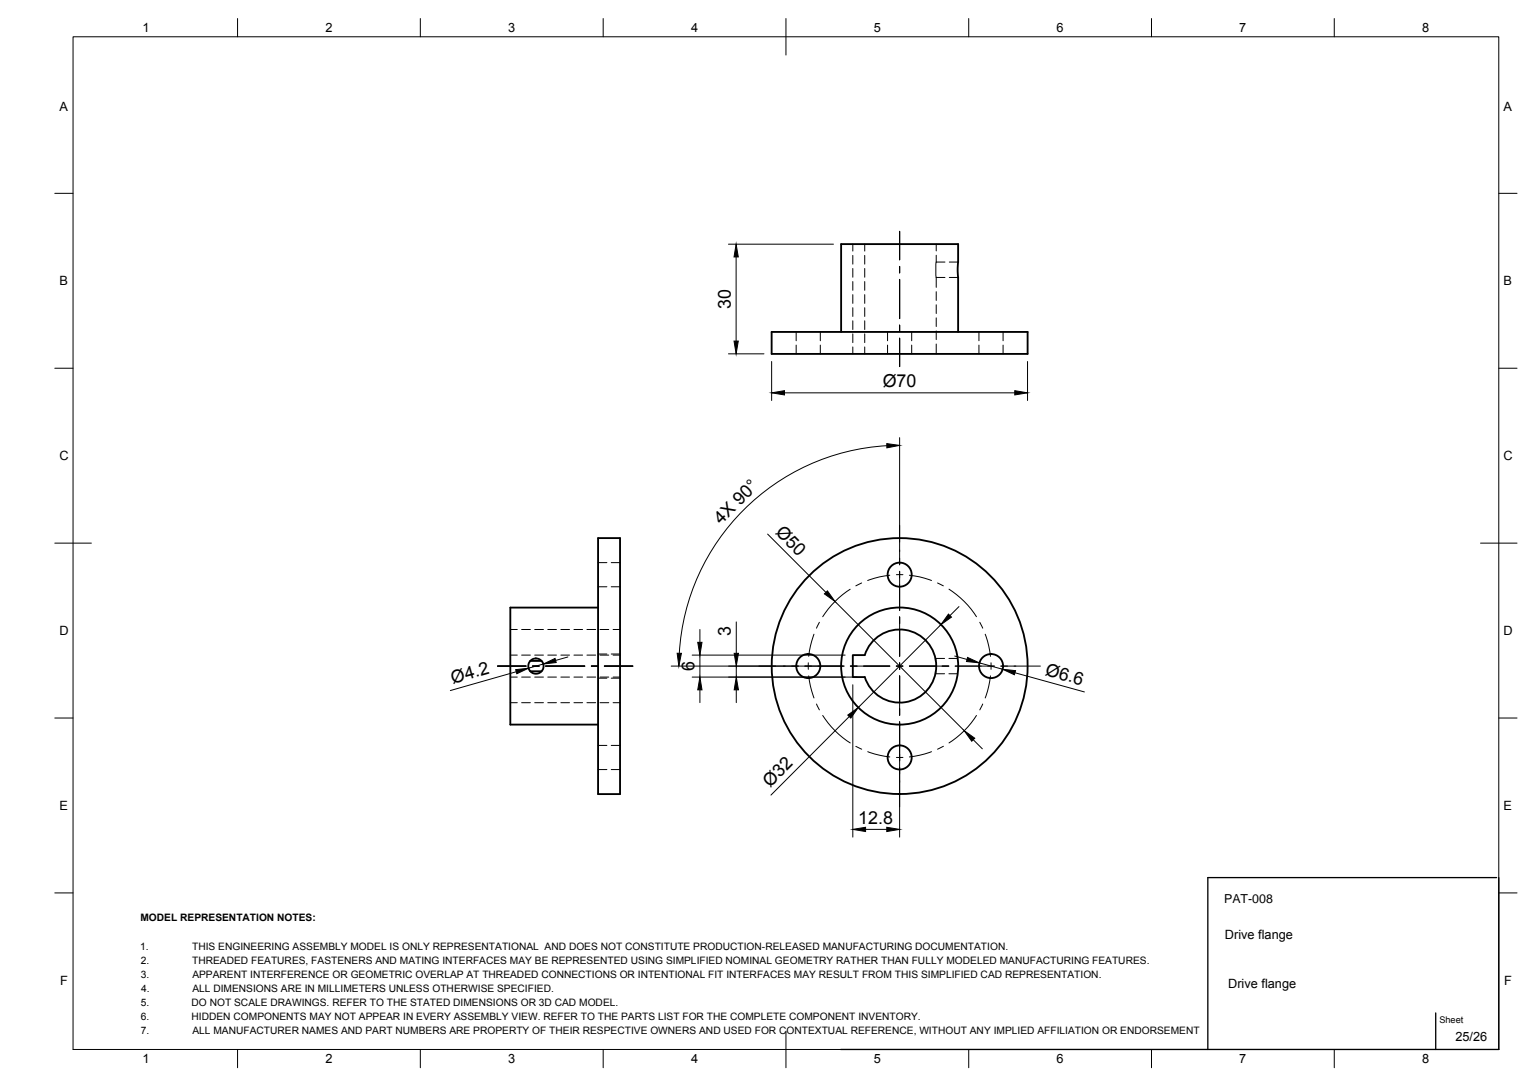
ISO-10303-21;
HEADER;
/* Generated by software containing ST-Developer
 * from STEP Tools, Inc. (www.steptools.com) 
 */

FILE_DESCRIPTION(
/* description */ ('Bearing housing with oil seal and end cap'),
/* implementation_level */ '2;1');

FILE_NAME(
/* name */ 'Drive flange.step',
/* time_stamp */ '2026-10-28T03:23:10-07:00',
/* author */ (''),
/* organization */ (''),
/* preprocessor_version */ 'ST-DEVELOPER v20.2',
/* originating_system */ 'Autodesk Translation Framework v15.17.0.0',
/* authorisation */ '');

FILE_SCHEMA (('AUTOMOTIVE_DESIGN { 1 0 10303 214 3 1 1 }'));
ENDSEC;

DATA;
#10=MECHANICAL_DESIGN_GEOMETRIC_PRESENTATION_REPRESENTATION('',(#285),#7871);
#181=B_SPLINE_CURVE_WITH_KNOTS('',3,(#7578,#7579,#7580,#7581,#7582,#7583,
#7584,#7585,#7586,#7587),.UNSPECIFIED.,.F.,.F.,(4,2,2,2,4),(0.803821788694075,
0.872950991853619,0.952307212900969,1.03166343394832,1.10079263710786),
 .UNSPECIFIED.);
#182=B_SPLINE_CURVE_WITH_KNOTS('',3,(#7593,#7594,#7595,#7596,#7597,#7598,
#7599,#7600,#7601,#7602,#7603,#7604,#7605,#7606,#7607,#7608,#7609,#7610),
 .UNSPECIFIED.,.F.,.F.,(4,2,2,2,2,2,2,2,4),(0.,0.0792028026112439,0.158405605222488,
0.237607602356377,0.316809599490266,0.396011596624156,0.475213593758045,
0.554416396369289,0.633619198980533),.UNSPECIFIED.);
#183=B_SPLINE_CURVE_WITH_KNOTS('',3,(#7611,#7612,#7613,#7614,#7615,#7616,
#7617,#7618,#7619,#7620,#7621,#7622,#7623,#7624,#7625,#7626,#7627,#7628),
 .UNSPECIFIED.,.F.,.F.,(4,2,2,2,2,2,2,2,4),(0.633619198980533,0.712822001591777,
0.792024804203021,0.87122680133691,0.9504287984708,1.02963079560469,1.10883279273858,
1.18803559534982,1.26723839796107),.UNSPECIFIED.);
#184=B_SPLINE_CURVE_WITH_KNOTS('',3,(#7631,#7632,#7633,#7634,#7635,#7636,
#7637,#7638,#7639,#7640),.UNSPECIFIED.,.F.,.F.,(4,2,2,2,4),(0.168950313426762,
0.238079516586307,0.317435737633656,0.396791958681006,0.465921161840551),
 .UNSPECIFIED.);
#235=SHAPE_REPRESENTATION_RELATIONSHIP('SRR','None',#7984,#256);
#256=ADVANCED_BREP_SHAPE_REPRESENTATION('',(#312),#7868);
#285=STYLED_ITEM('',(#8146),#312);
#312=MANIFOLD_SOLID_BREP('Body1',#4113);
#394=FACE_BOUND('',#1102,.T.);
#395=FACE_BOUND('',#1104,.T.);
#396=FACE_BOUND('',#1110,.T.);
#397=FACE_BOUND('',#1111,.T.);
#398=FACE_BOUND('',#1112,.T.);
#399=FACE_BOUND('',#1113,.T.);
#400=FACE_BOUND('',#1114,.T.);
#401=FACE_BOUND('',#1117,.T.);
#402=FACE_BOUND('',#1119,.T.);
#403=FACE_BOUND('',#1120,.T.);
#404=FACE_BOUND('',#1121,.T.);
#405=FACE_BOUND('',#1122,.T.);
#406=FACE_BOUND('',#1123,.T.);
#525=PLANE('',#4810);
#526=PLANE('',#4815);
#527=PLANE('',#4816);
#528=PLANE('',#4817);
#529=PLANE('',#4818);
#530=PLANE('',#4819);
#531=PLANE('',#4836);
#532=PLANE('',#4842);
#765=FACE_OUTER_BOUND('',#1095,.T.);
#766=FACE_OUTER_BOUND('',#1096,.T.);
#767=FACE_OUTER_BOUND('',#1097,.T.);
#768=FACE_OUTER_BOUND('',#1098,.T.);
#769=FACE_OUTER_BOUND('',#1099,.T.);
#770=FACE_OUTER_BOUND('',#1100,.T.);
#771=FACE_OUTER_BOUND('',#1101,.T.);
#772=FACE_OUTER_BOUND('',#1103,.T.);
#773=FACE_OUTER_BOUND('',#1105,.T.);
#774=FACE_OUTER_BOUND('',#1106,.T.);
#775=FACE_OUTER_BOUND('',#1107,.T.);
#776=FACE_OUTER_BOUND('',#1108,.T.);
#777=FACE_OUTER_BOUND('',#1109,.T.);
#778=FACE_OUTER_BOUND('',#1115,.T.);
#779=FACE_OUTER_BOUND('',#1116,.T.);
#780=FACE_OUTER_BOUND('',#1118,.T.);
#1095=EDGE_LOOP('',(#3581,#3582));
#1096=EDGE_LOOP('',(#3583,#3584,#3585,#3586,#3587,#3588,#3589,#3590,#3591));
#1097=EDGE_LOOP('',(#3592,#3593,#3594));
#1098=EDGE_LOOP('',(#3595,#3596,#3597,#3598));
#1099=EDGE_LOOP('',(#3599,#3600,#3601,#3602));
#1100=EDGE_LOOP('',(#3603,#3604,#3605,#3606));
#1101=EDGE_LOOP('',(#3607));
#1102=EDGE_LOOP('',(#3608,#3609,#3610,#3611));
#1103=EDGE_LOOP('',(#3612,#3613,#3614,#3615));
#1104=EDGE_LOOP('',(#3616,#3617,#3618,#3619));
#1105=EDGE_LOOP('',(#3620,#3621,#3622,#3623));
#1106=EDGE_LOOP('',(#3624,#3625,#3626,#3627));
#1107=EDGE_LOOP('',(#3628,#3629,#3630,#3631));
#1108=EDGE_LOOP('',(#3632,#3633,#3634,#3635));
#1109=EDGE_LOOP('',(#3636));
#1110=EDGE_LOOP('',(#3637));
#1111=EDGE_LOOP('',(#3638));
#1112=EDGE_LOOP('',(#3639));
#1113=EDGE_LOOP('',(#3640));
#1114=EDGE_LOOP('',(#3641));
#1115=EDGE_LOOP('',(#3642,#3643,#3644,#3645));
#1116=EDGE_LOOP('',(#3646,#3647,#3648,#3649));
#1117=EDGE_LOOP('',(#3650,#3651));
#1118=EDGE_LOOP('',(#3652));
#1119=EDGE_LOOP('',(#3653,#3654,#3655,#3656));
#1120=EDGE_LOOP('',(#3657));
#1121=EDGE_LOOP('',(#3658));
#1122=EDGE_LOOP('',(#3659));
#1123=EDGE_LOOP('',(#3660));
#1345=LINE('',#7574,#1607);
#1346=LINE('',#7591,#1608);
#1347=LINE('',#7642,#1609);
#1348=LINE('',#7646,#1610);
#1349=LINE('',#7648,#1611);
#1350=LINE('',#7650,#1612);
#1351=LINE('',#7651,#1613);
#1352=LINE('',#7654,#1614);
#1353=LINE('',#7656,#1615);
#1354=LINE('',#7657,#1616);
#1355=LINE('',#7660,#1617);
#1356=LINE('',#7662,#1618);
#1357=LINE('',#7663,#1619);
#1358=LINE('',#7674,#1620);
#1359=LINE('',#7680,#1621);
#1360=LINE('',#7686,#1622);
#1361=LINE('',#7692,#1623);
#1362=LINE('',#7701,#1624);
#1363=LINE('',#7704,#1625);
#1607=VECTOR('',#6004,1.);
#1608=VECTOR('',#6011,0.21);
#1609=VECTOR('',#6016,1.);
#1610=VECTOR('',#6019,1.);
#1611=VECTOR('',#6020,1.);
#1612=VECTOR('',#6021,1.);
#1613=VECTOR('',#6022,1.);
#1614=VECTOR('',#6025,1.);
#1615=VECTOR('',#6026,1.);
#1616=VECTOR('',#6027,1.);
#1617=VECTOR('',#6030,1.);
#1618=VECTOR('',#6031,1.);
#1619=VECTOR('',#6032,1.);
#1620=VECTOR('',#6047,0.33);
#1621=VECTOR('',#6054,0.33);
#1622=VECTOR('',#6061,0.33);
#1623=VECTOR('',#6068,0.33);
#1624=VECTOR('',#6079,3.5);
#1625=VECTOR('',#6084,1.6);
#1870=CIRCLE('',#4811,0.21);
#1871=CIRCLE('',#4813,0.21);
#1872=CIRCLE('',#4814,0.21);
#1873=CIRCLE('',#4820,1.6);
#1874=CIRCLE('',#4821,1.);
#1875=CIRCLE('',#4823,1.);
#1876=CIRCLE('',#4825,0.33);
#1877=CIRCLE('',#4826,0.33);
#1878=CIRCLE('',#4828,0.33);
#1879=CIRCLE('',#4829,0.33);
#1880=CIRCLE('',#4831,0.33);
#1881=CIRCLE('',#4832,0.33);
#1882=CIRCLE('',#4834,0.33);
#1883=CIRCLE('',#4835,0.33);
#1884=CIRCLE('',#4837,3.5);
#1885=CIRCLE('',#4838,1.6);
#1886=CIRCLE('',#4840,3.5);
#2176=VERTEX_POINT('',#7572);
#2177=VERTEX_POINT('',#7573);
#2178=VERTEX_POINT('',#7577);
#2179=VERTEX_POINT('',#7588);
#2180=VERTEX_POINT('',#7590);
#2181=VERTEX_POINT('',#7592);
#2182=VERTEX_POINT('',#7629);
#2183=VERTEX_POINT('',#7644);
#2184=VERTEX_POINT('',#7645);
#2185=VERTEX_POINT('',#7647);
#2186=VERTEX_POINT('',#7649);
#2187=VERTEX_POINT('',#7653);
#2188=VERTEX_POINT('',#7655);
#2189=VERTEX_POINT('',#7659);
#2190=VERTEX_POINT('',#7661);
#2191=VERTEX_POINT('',#7665);
#2192=VERTEX_POINT('',#7671);
#2193=VERTEX_POINT('',#7673);
#2194=VERTEX_POINT('',#7677);
#2195=VERTEX_POINT('',#7679);
#2196=VERTEX_POINT('',#7683);
#2197=VERTEX_POINT('',#7685);
#2198=VERTEX_POINT('',#7689);
#2199=VERTEX_POINT('',#7691);
#2200=VERTEX_POINT('',#7695);
#2201=VERTEX_POINT('',#7697);
#2202=VERTEX_POINT('',#7700);
#2654=EDGE_CURVE('',#2176,#2177,#1345,.T.);
#2655=EDGE_CURVE('',#2176,#2177,#1870,.T.);
#2656=EDGE_CURVE('',#2178,#2176,#181,.T.);
#2657=EDGE_CURVE('',#2179,#2178,#1871,.T.);
#2658=EDGE_CURVE('',#2179,#2180,#1346,.T.);
#2659=EDGE_CURVE('',#2181,#2180,#182,.T.);
#2660=EDGE_CURVE('',#2180,#2181,#183,.T.);
#2661=EDGE_CURVE('',#2182,#2179,#1872,.T.);
#2662=EDGE_CURVE('',#2177,#2182,#184,.T.);
#2663=EDGE_CURVE('',#2182,#2178,#1347,.T.);
#2664=EDGE_CURVE('',#2183,#2184,#1348,.T.);
#2665=EDGE_CURVE('',#2183,#2185,#1349,.T.);
#2666=EDGE_CURVE('',#2186,#2185,#1350,.T.);
#2667=EDGE_CURVE('',#2184,#2186,#1351,.T.);
#2668=EDGE_CURVE('',#2187,#2183,#1352,.T.);
#2669=EDGE_CURVE('',#2187,#2188,#1353,.T.);
#2670=EDGE_CURVE('',#2185,#2188,#1354,.T.);
#2671=EDGE_CURVE('',#2189,#2187,#1355,.T.);
#2672=EDGE_CURVE('',#2190,#2189,#1356,.T.);
#2673=EDGE_CURVE('',#2188,#2190,#1357,.T.);
#2674=EDGE_CURVE('',#2191,#2191,#1873,.T.);
#2675=EDGE_CURVE('',#2190,#2186,#1874,.T.);
#2676=EDGE_CURVE('',#2189,#2184,#1875,.T.);
#2677=EDGE_CURVE('',#2192,#2192,#1876,.T.);
#2678=EDGE_CURVE('',#2192,#2193,#1358,.T.);
#2679=EDGE_CURVE('',#2193,#2193,#1877,.T.);
#2680=EDGE_CURVE('',#2194,#2194,#1878,.T.);
#2681=EDGE_CURVE('',#2194,#2195,#1359,.T.);
#2682=EDGE_CURVE('',#2195,#2195,#1879,.T.);
#2683=EDGE_CURVE('',#2196,#2196,#1880,.T.);
#2684=EDGE_CURVE('',#2196,#2197,#1360,.T.);
#2685=EDGE_CURVE('',#2197,#2197,#1881,.T.);
#2686=EDGE_CURVE('',#2198,#2198,#1882,.T.);
#2687=EDGE_CURVE('',#2198,#2199,#1361,.T.);
#2688=EDGE_CURVE('',#2199,#2199,#1883,.T.);
#2689=EDGE_CURVE('',#2200,#2200,#1884,.T.);
#2690=EDGE_CURVE('',#2201,#2201,#1885,.T.);
#2691=EDGE_CURVE('',#2200,#2202,#1362,.T.);
#2692=EDGE_CURVE('',#2202,#2202,#1886,.T.);
#2693=EDGE_CURVE('',#2191,#2201,#1363,.T.);
#3581=ORIENTED_EDGE('',*,*,#2654,.F.);
#3582=ORIENTED_EDGE('',*,*,#2655,.T.);
#3583=ORIENTED_EDGE('',*,*,#2656,.F.);
#3584=ORIENTED_EDGE('',*,*,#2657,.F.);
#3585=ORIENTED_EDGE('',*,*,#2658,.T.);
#3586=ORIENTED_EDGE('',*,*,#2659,.F.);
#3587=ORIENTED_EDGE('',*,*,#2660,.F.);
#3588=ORIENTED_EDGE('',*,*,#2658,.F.);
#3589=ORIENTED_EDGE('',*,*,#2661,.F.);
#3590=ORIENTED_EDGE('',*,*,#2662,.F.);
#3591=ORIENTED_EDGE('',*,*,#2655,.F.);
#3592=ORIENTED_EDGE('',*,*,#2663,.F.);
#3593=ORIENTED_EDGE('',*,*,#2661,.T.);
#3594=ORIENTED_EDGE('',*,*,#2657,.T.);
#3595=ORIENTED_EDGE('',*,*,#2664,.F.);
#3596=ORIENTED_EDGE('',*,*,#2665,.T.);
#3597=ORIENTED_EDGE('',*,*,#2666,.F.);
#3598=ORIENTED_EDGE('',*,*,#2667,.F.);
#3599=ORIENTED_EDGE('',*,*,#2668,.F.);
#3600=ORIENTED_EDGE('',*,*,#2669,.T.);
#3601=ORIENTED_EDGE('',*,*,#2670,.F.);
#3602=ORIENTED_EDGE('',*,*,#2665,.F.);
#3603=ORIENTED_EDGE('',*,*,#2671,.F.);
#3604=ORIENTED_EDGE('',*,*,#2672,.F.);
#3605=ORIENTED_EDGE('',*,*,#2673,.F.);
#3606=ORIENTED_EDGE('',*,*,#2669,.F.);
#3607=ORIENTED_EDGE('',*,*,#2674,.T.);
#3608=ORIENTED_EDGE('',*,*,#2666,.T.);
#3609=ORIENTED_EDGE('',*,*,#2670,.T.);
#3610=ORIENTED_EDGE('',*,*,#2673,.T.);
#3611=ORIENTED_EDGE('',*,*,#2675,.T.);
#3612=ORIENTED_EDGE('',*,*,#2667,.T.);
#3613=ORIENTED_EDGE('',*,*,#2675,.F.);
#3614=ORIENTED_EDGE('',*,*,#2672,.T.);
#3615=ORIENTED_EDGE('',*,*,#2676,.T.);
#3616=ORIENTED_EDGE('',*,*,#2662,.T.);
#3617=ORIENTED_EDGE('',*,*,#2663,.T.);
#3618=ORIENTED_EDGE('',*,*,#2656,.T.);
#3619=ORIENTED_EDGE('',*,*,#2654,.T.);
#3620=ORIENTED_EDGE('',*,*,#2677,.F.);
#3621=ORIENTED_EDGE('',*,*,#2678,.T.);
#3622=ORIENTED_EDGE('',*,*,#2679,.F.);
#3623=ORIENTED_EDGE('',*,*,#2678,.F.);
#3624=ORIENTED_EDGE('',*,*,#2680,.F.);
#3625=ORIENTED_EDGE('',*,*,#2681,.T.);
#3626=ORIENTED_EDGE('',*,*,#2682,.F.);
#3627=ORIENTED_EDGE('',*,*,#2681,.F.);
#3628=ORIENTED_EDGE('',*,*,#2683,.F.);
#3629=ORIENTED_EDGE('',*,*,#2684,.T.);
#3630=ORIENTED_EDGE('',*,*,#2685,.F.);
#3631=ORIENTED_EDGE('',*,*,#2684,.F.);
#3632=ORIENTED_EDGE('',*,*,#2686,.F.);
#3633=ORIENTED_EDGE('',*,*,#2687,.T.);
#3634=ORIENTED_EDGE('',*,*,#2688,.F.);
#3635=ORIENTED_EDGE('',*,*,#2687,.F.);
#3636=ORIENTED_EDGE('',*,*,#2689,.T.);
#3637=ORIENTED_EDGE('',*,*,#2690,.F.);
#3638=ORIENTED_EDGE('',*,*,#2688,.T.);
#3639=ORIENTED_EDGE('',*,*,#2685,.T.);
#3640=ORIENTED_EDGE('',*,*,#2682,.T.);
#3641=ORIENTED_EDGE('',*,*,#2679,.T.);
#3642=ORIENTED_EDGE('',*,*,#2689,.F.);
#3643=ORIENTED_EDGE('',*,*,#2691,.T.);
#3644=ORIENTED_EDGE('',*,*,#2692,.T.);
#3645=ORIENTED_EDGE('',*,*,#2691,.F.);
#3646=ORIENTED_EDGE('',*,*,#2674,.F.);
#3647=ORIENTED_EDGE('',*,*,#2693,.T.);
#3648=ORIENTED_EDGE('',*,*,#2690,.T.);
#3649=ORIENTED_EDGE('',*,*,#2693,.F.);
#3650=ORIENTED_EDGE('',*,*,#2659,.T.);
#3651=ORIENTED_EDGE('',*,*,#2660,.T.);
#3652=ORIENTED_EDGE('',*,*,#2692,.F.);
#3653=ORIENTED_EDGE('',*,*,#2664,.T.);
#3654=ORIENTED_EDGE('',*,*,#2676,.F.);
#3655=ORIENTED_EDGE('',*,*,#2671,.T.);
#3656=ORIENTED_EDGE('',*,*,#2668,.T.);
#3657=ORIENTED_EDGE('',*,*,#2686,.T.);
#3658=ORIENTED_EDGE('',*,*,#2683,.T.);
#3659=ORIENTED_EDGE('',*,*,#2680,.T.);
#3660=ORIENTED_EDGE('',*,*,#2677,.T.);
#3825=CYLINDRICAL_SURFACE('',#4812,0.21);
#3826=CYLINDRICAL_SURFACE('',#4822,1.);
#3827=CYLINDRICAL_SURFACE('',#4824,0.33);
#3828=CYLINDRICAL_SURFACE('',#4827,0.33);
#3829=CYLINDRICAL_SURFACE('',#4830,0.33);
#3830=CYLINDRICAL_SURFACE('',#4833,0.33);
#3831=CYLINDRICAL_SURFACE('',#4839,3.5);
#3832=CYLINDRICAL_SURFACE('',#4841,1.6);
#4047=ADVANCED_FACE('',(#765),#525,.T.);
#4048=ADVANCED_FACE('',(#766),#3825,.F.);
#4049=ADVANCED_FACE('',(#767),#526,.T.);
#4050=ADVANCED_FACE('',(#768),#527,.F.);
#4051=ADVANCED_FACE('',(#769),#528,.F.);
#4052=ADVANCED_FACE('',(#770),#529,.F.);
#4053=ADVANCED_FACE('',(#771,#394),#530,.T.);
#4054=ADVANCED_FACE('',(#772,#395),#3826,.F.);
#4055=ADVANCED_FACE('',(#773),#3827,.F.);
#4056=ADVANCED_FACE('',(#774),#3828,.F.);
#4057=ADVANCED_FACE('',(#775),#3829,.F.);
#4058=ADVANCED_FACE('',(#776),#3830,.F.);
#4059=ADVANCED_FACE('',(#777,#396,#397,#398,#399,#400),#531,.T.);
#4060=ADVANCED_FACE('',(#778),#3831,.T.);
#4061=ADVANCED_FACE('',(#779,#401),#3832,.T.);
#4062=ADVANCED_FACE('',(#780,#402,#403,#404,#405,#406),#532,.F.);
#4113=CLOSED_SHELL('',(#4047,#4048,#4049,#4050,#4051,#4052,#4053,#4054,
#4055,#4056,#4057,#4058,#4059,#4060,#4061,#4062));
#4809=AXIS2_PLACEMENT_3D('',#7570,#6000,#6001);
#4810=AXIS2_PLACEMENT_3D('',#7571,#6002,#6003);
#4811=AXIS2_PLACEMENT_3D('',#7575,#6005,#6006);
#4812=AXIS2_PLACEMENT_3D('',#7576,#6007,#6008);
#4813=AXIS2_PLACEMENT_3D('',#7589,#6009,#6010);
#4814=AXIS2_PLACEMENT_3D('',#7630,#6012,#6013);
#4815=AXIS2_PLACEMENT_3D('',#7641,#6014,#6015);
#4816=AXIS2_PLACEMENT_3D('',#7643,#6017,#6018);
#4817=AXIS2_PLACEMENT_3D('',#7652,#6023,#6024);
#4818=AXIS2_PLACEMENT_3D('',#7658,#6028,#6029);
#4819=AXIS2_PLACEMENT_3D('',#7664,#6033,#6034);
#4820=AXIS2_PLACEMENT_3D('',#7666,#6035,#6036);
#4821=AXIS2_PLACEMENT_3D('',#7667,#6037,#6038);
#4822=AXIS2_PLACEMENT_3D('',#7668,#6039,#6040);
#4823=AXIS2_PLACEMENT_3D('',#7669,#6041,#6042);
#4824=AXIS2_PLACEMENT_3D('',#7670,#6043,#6044);
#4825=AXIS2_PLACEMENT_3D('',#7672,#6045,#6046);
#4826=AXIS2_PLACEMENT_3D('',#7675,#6048,#6049);
#4827=AXIS2_PLACEMENT_3D('',#7676,#6050,#6051);
#4828=AXIS2_PLACEMENT_3D('',#7678,#6052,#6053);
#4829=AXIS2_PLACEMENT_3D('',#7681,#6055,#6056);
#4830=AXIS2_PLACEMENT_3D('',#7682,#6057,#6058);
#4831=AXIS2_PLACEMENT_3D('',#7684,#6059,#6060);
#4832=AXIS2_PLACEMENT_3D('',#7687,#6062,#6063);
#4833=AXIS2_PLACEMENT_3D('',#7688,#6064,#6065);
#4834=AXIS2_PLACEMENT_3D('',#7690,#6066,#6067);
#4835=AXIS2_PLACEMENT_3D('',#7693,#6069,#6070);
#4836=AXIS2_PLACEMENT_3D('',#7694,#6071,#6072);
#4837=AXIS2_PLACEMENT_3D('',#7696,#6073,#6074);
#4838=AXIS2_PLACEMENT_3D('',#7698,#6075,#6076);
#4839=AXIS2_PLACEMENT_3D('',#7699,#6077,#6078);
#4840=AXIS2_PLACEMENT_3D('',#7702,#6080,#6081);
#4841=AXIS2_PLACEMENT_3D('',#7703,#6082,#6083);
#4842=AXIS2_PLACEMENT_3D('',#7705,#6085,#6086);
#6000=DIRECTION('axis',(0.,0.,1.));
#6001=DIRECTION('refdir',(1.,0.,0.));
#6002=DIRECTION('center_axis',(0.,0.,1.));
#6003=DIRECTION('ref_axis',(1.,0.,0.));
#6004=DIRECTION('',(0.,1.,0.));
#6005=DIRECTION('center_axis',(0.,0.,1.));
#6006=DIRECTION('ref_axis',(1.,0.,0.));
#6007=DIRECTION('center_axis',(0.,0.,1.));
#6008=DIRECTION('ref_axis',(1.,0.,0.));
#6009=DIRECTION('center_axis',(0.,0.,1.));
#6010=DIRECTION('ref_axis',(1.,0.,0.));
#6011=DIRECTION('',(0.,0.,1.));
#6012=DIRECTION('center_axis',(0.,0.,1.));
#6013=DIRECTION('ref_axis',(1.,0.,0.));
#6014=DIRECTION('center_axis',(0.,0.,1.));
#6015=DIRECTION('ref_axis',(1.,0.,0.));
#6016=DIRECTION('',(0.,-1.,0.));
#6017=DIRECTION('center_axis',(-1.,0.,0.));
#6018=DIRECTION('ref_axis',(0.,0.,1.));
#6019=DIRECTION('',(0.,0.,1.));
#6020=DIRECTION('',(0.,1.,0.));
#6021=DIRECTION('',(0.,0.,-1.));
#6022=DIRECTION('',(0.,1.,0.));
#6023=DIRECTION('center_axis',(0.,0.,-1.));
#6024=DIRECTION('ref_axis',(-1.,0.,0.));
#6025=DIRECTION('',(-1.,0.,0.));
#6026=DIRECTION('',(0.,1.,0.));
#6027=DIRECTION('',(1.,0.,0.));
#6028=DIRECTION('center_axis',(1.,0.,0.));
#6029=DIRECTION('ref_axis',(0.,0.,-1.));
#6030=DIRECTION('',(0.,0.,-1.));
#6031=DIRECTION('',(0.,-1.,0.));
#6032=DIRECTION('',(0.,0.,1.));
#6033=DIRECTION('center_axis',(0.,1.,0.));
#6034=DIRECTION('ref_axis',(1.,0.,0.));
#6035=DIRECTION('center_axis',(0.,1.,0.));
#6036=DIRECTION('ref_axis',(1.,0.,0.));
#6037=DIRECTION('center_axis',(0.,-1.,0.));
#6038=DIRECTION('ref_axis',(1.,0.,0.));
#6039=DIRECTION('center_axis',(0.,1.,0.));
#6040=DIRECTION('ref_axis',(-1.83697019872103E-16,0.,1.));
#6041=DIRECTION('center_axis',(0.,-1.,0.));
#6042=DIRECTION('ref_axis',(1.,0.,0.));
#6043=DIRECTION('center_axis',(0.,1.,0.));
#6044=DIRECTION('ref_axis',(1.,0.,0.));
#6045=DIRECTION('center_axis',(0.,1.,0.));
#6046=DIRECTION('ref_axis',(1.,0.,0.));
#6047=DIRECTION('',(0.,1.,0.));
#6048=DIRECTION('center_axis',(0.,-1.,0.));
#6049=DIRECTION('ref_axis',(1.,0.,0.));
#6050=DIRECTION('center_axis',(0.,1.,0.));
#6051=DIRECTION('ref_axis',(1.,0.,0.));
#6052=DIRECTION('center_axis',(0.,1.,0.));
#6053=DIRECTION('ref_axis',(1.,0.,0.));
#6054=DIRECTION('',(0.,1.,0.));
#6055=DIRECTION('center_axis',(0.,-1.,0.));
#6056=DIRECTION('ref_axis',(1.,0.,0.));
#6057=DIRECTION('center_axis',(0.,1.,0.));
#6058=DIRECTION('ref_axis',(1.,0.,0.));
#6059=DIRECTION('center_axis',(0.,1.,0.));
#6060=DIRECTION('ref_axis',(1.,0.,0.));
#6061=DIRECTION('',(0.,1.,0.));
#6062=DIRECTION('center_axis',(0.,-1.,0.));
#6063=DIRECTION('ref_axis',(1.,0.,0.));
#6064=DIRECTION('center_axis',(0.,1.,0.));
#6065=DIRECTION('ref_axis',(1.,0.,0.));
#6066=DIRECTION('center_axis',(0.,1.,0.));
#6067=DIRECTION('ref_axis',(1.,0.,0.));
#6068=DIRECTION('',(0.,1.,0.));
#6069=DIRECTION('center_axis',(0.,-1.,0.));
#6070=DIRECTION('ref_axis',(1.,0.,0.));
#6071=DIRECTION('center_axis',(0.,1.,0.));
#6072=DIRECTION('ref_axis',(1.,0.,0.));
#6073=DIRECTION('center_axis',(0.,1.,0.));
#6074=DIRECTION('ref_axis',(1.,0.,0.));
#6075=DIRECTION('center_axis',(0.,1.,0.));
#6076=DIRECTION('ref_axis',(1.,0.,0.));
#6077=DIRECTION('center_axis',(0.,1.,0.));
#6078=DIRECTION('ref_axis',(1.,0.,0.));
#6079=DIRECTION('',(0.,-1.,0.));
#6080=DIRECTION('center_axis',(0.,1.,0.));
#6081=DIRECTION('ref_axis',(1.,0.,0.));
#6082=DIRECTION('center_axis',(0.,1.,0.));
#6083=DIRECTION('ref_axis',(1.,0.,0.));
#6084=DIRECTION('',(0.,-1.,0.));
#6085=DIRECTION('center_axis',(0.,1.,0.));
#6086=DIRECTION('ref_axis',(1.,0.,0.));
#7570=CARTESIAN_POINT('',(0.,0.,0.));
#7571=CARTESIAN_POINT('Origin',(0.,-1.2,5.49));
#7572=CARTESIAN_POINT('',(0.141067359796657,-1.35556349186104,5.49));
#7573=CARTESIAN_POINT('',(0.141067359796657,-1.04443650813896,5.49));
#7574=CARTESIAN_POINT('',(0.141067359796657,-3.5,5.49));
#7575=CARTESIAN_POINT('Origin',(0.,-1.2,5.49));
#7576=CARTESIAN_POINT('Origin',(0.,-1.2,5.49));
#7577=CARTESIAN_POINT('',(-0.141067359796657,-1.35556349186104,5.49));
#7578=CARTESIAN_POINT('Ctrl Pts',(-0.141067359796657,-1.35556349186104,
5.49));
#7579=CARTESIAN_POINT('Ctrl Pts',(-0.123818356698224,-1.3712051523632,5.49245784982446));
#7580=CARTESIAN_POINT('Ctrl Pts',(-0.102998643109699,-1.38462404333102,
5.49493819304946));
#7581=CARTESIAN_POINT('Ctrl Pts',(-0.054614114398353,-1.40469746372443,
5.49884449237241));
#7582=CARTESIAN_POINT('Ctrl Pts',(-0.0264520736824499,-1.41,5.5));
#7583=CARTESIAN_POINT('Ctrl Pts',(0.0264520736824498,-1.41,5.5));
#7584=CARTESIAN_POINT('Ctrl Pts',(0.0546141143983528,-1.40469746372443,
5.49884449237241));
#7585=CARTESIAN_POINT('Ctrl Pts',(0.102998643109699,-1.38462404333102,5.49493819304946));
#7586=CARTESIAN_POINT('Ctrl Pts',(0.123818356698224,-1.3712051523632,5.49245784982446));
#7587=CARTESIAN_POINT('Ctrl Pts',(0.141067359796657,-1.35556349186104,5.49));
#7588=CARTESIAN_POINT('',(-0.21,-1.2,5.49));
#7589=CARTESIAN_POINT('Origin',(0.,-1.2,5.49));
#7590=CARTESIAN_POINT('',(-0.21,-1.2,6.08615888233178));
#7591=CARTESIAN_POINT('',(-0.21,-1.2,5.49));
#7592=CARTESIAN_POINT('',(0.21,-1.2,6.08615888233178));
#7593=CARTESIAN_POINT('Ctrl Pts',(0.21,-1.2,6.08615888233178));
#7594=CARTESIAN_POINT('Ctrl Pts',(0.21,-1.22640093420375,6.08615888233178));
#7595=CARTESIAN_POINT('Ctrl Pts',(0.20471752266132,-1.25454055536511,6.08688606295397));
#7596=CARTESIAN_POINT('Ctrl Pts',(0.183276841782292,-1.3062710523005,6.08950502964782));
#7597=CARTESIAN_POINT('Ctrl Pts',(0.167120287247804,-1.32986456085055,6.09135816887013));
#7598=CARTESIAN_POINT('Ctrl Pts',(0.129864750292352,-1.367120097806,6.09483075953278));
#7599=CARTESIAN_POINT('Ctrl Pts',(0.106271159541076,-1.38327680083123,6.09667690933009));
#7600=CARTESIAN_POINT('Ctrl Pts',(0.0545403836274685,-1.4047175903444,6.09927985626981));
#7601=CARTESIAN_POINT('Ctrl Pts',(0.0264006657112964,-1.41,6.1));
#7602=CARTESIAN_POINT('Ctrl Pts',(-0.0264006657112964,-1.41,6.1));
#7603=CARTESIAN_POINT('Ctrl Pts',(-0.0545403836274684,-1.4047175903444,
6.09927985626981));
#7604=CARTESIAN_POINT('Ctrl Pts',(-0.106271159541075,-1.38327680083123,
6.09667690933009));
#7605=CARTESIAN_POINT('Ctrl Pts',(-0.129864750292352,-1.367120097806,6.09483075953278));
#7606=CARTESIAN_POINT('Ctrl Pts',(-0.167120287247804,-1.32986456085055,
6.09135816887013));
#7607=CARTESIAN_POINT('Ctrl Pts',(-0.183276841782292,-1.3062710523005,6.08950502964782));
#7608=CARTESIAN_POINT('Ctrl Pts',(-0.20471752266132,-1.25454055536511,6.08688606295397));
#7609=CARTESIAN_POINT('Ctrl Pts',(-0.21,-1.22640093420375,6.08615888233178));
#7610=CARTESIAN_POINT('Ctrl Pts',(-0.21,-1.2,6.08615888233178));
#7611=CARTESIAN_POINT('Ctrl Pts',(-0.21,-1.2,6.08615888233178));
#7612=CARTESIAN_POINT('Ctrl Pts',(-0.21,-1.17359906579625,6.08615888233178));
#7613=CARTESIAN_POINT('Ctrl Pts',(-0.20471752266132,-1.14545944463489,6.08688606295397));
#7614=CARTESIAN_POINT('Ctrl Pts',(-0.183276841782292,-1.0937289476995,6.08950502964782));
#7615=CARTESIAN_POINT('Ctrl Pts',(-0.167120287247804,-1.07013543914945,
6.09135816887013));
#7616=CARTESIAN_POINT('Ctrl Pts',(-0.129864750292352,-1.032879902194,6.09483075953278));
#7617=CARTESIAN_POINT('Ctrl Pts',(-0.106271159541076,-1.01672319916877,
6.09667690933009));
#7618=CARTESIAN_POINT('Ctrl Pts',(-0.0545403836274687,-0.995282409655599,
6.09927985626981));
#7619=CARTESIAN_POINT('Ctrl Pts',(-0.0264006657112964,-0.99,6.1));
#7620=CARTESIAN_POINT('Ctrl Pts',(0.0264006657112964,-0.99,6.1));
#7621=CARTESIAN_POINT('Ctrl Pts',(0.0545403836274687,-0.995282409655599,
6.09927985626981));
#7622=CARTESIAN_POINT('Ctrl Pts',(0.106271159541076,-1.01672319916877,6.09667690933009));
#7623=CARTESIAN_POINT('Ctrl Pts',(0.129864750292352,-1.032879902194,6.09483075953278));
#7624=CARTESIAN_POINT('Ctrl Pts',(0.167120287247804,-1.07013543914945,6.09135816887013));
#7625=CARTESIAN_POINT('Ctrl Pts',(0.183276841782292,-1.0937289476995,6.08950502964782));
#7626=CARTESIAN_POINT('Ctrl Pts',(0.20471752266132,-1.14545944463489,6.08688606295397));
#7627=CARTESIAN_POINT('Ctrl Pts',(0.21,-1.17359906579625,6.08615888233178));
#7628=CARTESIAN_POINT('Ctrl Pts',(0.21,-1.2,6.08615888233178));
#7629=CARTESIAN_POINT('',(-0.141067359796657,-1.04443650813896,5.49));
#7630=CARTESIAN_POINT('Origin',(0.,-1.2,5.49));
#7631=CARTESIAN_POINT('Ctrl Pts',(0.141067359796657,-1.04443650813896,5.49));
#7632=CARTESIAN_POINT('Ctrl Pts',(0.123818356698224,-1.0287948476368,5.49245784982446));
#7633=CARTESIAN_POINT('Ctrl Pts',(0.102998643109699,-1.01537595666898,5.49493819304946));
#7634=CARTESIAN_POINT('Ctrl Pts',(0.0546141143983531,-0.995302536275572,
5.49884449237241));
#7635=CARTESIAN_POINT('Ctrl Pts',(0.0264520736824498,-0.99,5.5));
#7636=CARTESIAN_POINT('Ctrl Pts',(-0.0264520736824498,-0.99,5.5));
#7637=CARTESIAN_POINT('Ctrl Pts',(-0.054614114398353,-0.995302536275572,
5.49884449237241));
#7638=CARTESIAN_POINT('Ctrl Pts',(-0.102998643109699,-1.01537595666898,
5.49493819304946));
#7639=CARTESIAN_POINT('Ctrl Pts',(-0.123818356698224,-1.0287948476368,5.49245784982446));
#7640=CARTESIAN_POINT('Ctrl Pts',(-0.141067359796657,-1.04443650813896,
5.49));
#7641=CARTESIAN_POINT('Origin',(0.,-1.2,5.49));
#7642=CARTESIAN_POINT('',(-0.141067359796657,-3.5,5.49));
#7643=CARTESIAN_POINT('Origin',(-0.3,-3.6,3.22));
#7644=CARTESIAN_POINT('',(-0.3,-3.5,3.22));
#7645=CARTESIAN_POINT('',(-0.3,-3.5,3.54606079858305));
#7646=CARTESIAN_POINT('',(-0.3,-3.5,3.86));
#7647=CARTESIAN_POINT('',(-0.3,-0.5,3.22));
#7648=CARTESIAN_POINT('',(-0.3,-3.6,3.22));
#7649=CARTESIAN_POINT('',(-0.3,-0.5,3.54606079858305));
#7650=CARTESIAN_POINT('',(-0.3,-0.5,3.86));
#7651=CARTESIAN_POINT('',(-0.3,-3.5,3.54606079858305));
#7652=CARTESIAN_POINT('Origin',(0.3,-3.6,3.22));
#7653=CARTESIAN_POINT('',(0.3,-3.5,3.22));
#7654=CARTESIAN_POINT('',(0.15,-3.5,3.22));
#7655=CARTESIAN_POINT('',(0.3,-0.5,3.22));
#7656=CARTESIAN_POINT('',(0.3,-3.6,3.22));
#7657=CARTESIAN_POINT('',(0.15,-0.5,3.22));
#7658=CARTESIAN_POINT('Origin',(0.3,-3.6,4.5));
#7659=CARTESIAN_POINT('',(0.3,-3.5,3.54606079858305));
#7660=CARTESIAN_POINT('',(0.3,-3.5,4.5));
#7661=CARTESIAN_POINT('',(0.3,-0.5,3.54606079858305));
#7662=CARTESIAN_POINT('',(0.3,-3.5,3.54606079858305));
#7663=CARTESIAN_POINT('',(0.3,-0.5,4.5));
#7664=CARTESIAN_POINT('Origin',(0.,-0.5,4.5));
#7665=CARTESIAN_POINT('',(-1.6,-0.5,4.5));
#7666=CARTESIAN_POINT('Origin',(0.,-0.5,4.5));
#7667=CARTESIAN_POINT('Origin',(0.,-0.5,4.5));
#7668=CARTESIAN_POINT('Origin',(0.,-3.5,4.5));
#7669=CARTESIAN_POINT('Origin',(0.,-3.5,4.5));
#7670=CARTESIAN_POINT('Origin',(-2.5,-3.6,4.5));
#7671=CARTESIAN_POINT('',(-2.83,-3.5,4.5));
#7672=CARTESIAN_POINT('Origin',(-2.5,-3.5,4.5));
#7673=CARTESIAN_POINT('',(-2.83,-2.9,4.5));
#7674=CARTESIAN_POINT('',(-2.83,-3.6,4.5));
#7675=CARTESIAN_POINT('Origin',(-2.5,-2.9,4.5));
#7676=CARTESIAN_POINT('Origin',(1.53080849893419E-16,-3.6,7.));
#7677=CARTESIAN_POINT('',(-0.33,-3.5,7.));
#7678=CARTESIAN_POINT('Origin',(1.53080849893419E-16,-3.5,7.));
#7679=CARTESIAN_POINT('',(-0.33,-2.9,7.));
#7680=CARTESIAN_POINT('',(-0.33,-3.6,7.));
#7681=CARTESIAN_POINT('Origin',(1.53080849893419E-16,-2.9,7.));
#7682=CARTESIAN_POINT('Origin',(2.5,-3.6,4.5));
#7683=CARTESIAN_POINT('',(2.17,-3.5,4.5));
#7684=CARTESIAN_POINT('Origin',(2.5,-3.5,4.5));
#7685=CARTESIAN_POINT('',(2.17,-2.9,4.5));
#7686=CARTESIAN_POINT('',(2.17,-3.6,4.5));
#7687=CARTESIAN_POINT('Origin',(2.5,-2.9,4.5));
#7688=CARTESIAN_POINT('Origin',(-4.59242549680257E-16,-3.6,2.));
#7689=CARTESIAN_POINT('',(-0.33,-3.5,2.));
#7690=CARTESIAN_POINT('Origin',(-4.59242549680257E-16,-3.5,2.));
#7691=CARTESIAN_POINT('',(-0.33,-2.9,2.));
#7692=CARTESIAN_POINT('',(-0.33,-3.6,2.));
#7693=CARTESIAN_POINT('Origin',(-4.59242549680257E-16,-2.9,2.));
#7694=CARTESIAN_POINT('Origin',(0.,-2.9,4.5));
#7695=CARTESIAN_POINT('',(-3.5,-2.9,4.5));
#7696=CARTESIAN_POINT('Origin',(0.,-2.9,4.5));
#7697=CARTESIAN_POINT('',(-1.6,-2.9,4.5));
#7698=CARTESIAN_POINT('Origin',(0.,-2.9,4.5));
#7699=CARTESIAN_POINT('Origin',(0.,-3.5,4.5));
#7700=CARTESIAN_POINT('',(-3.5,-3.5,4.5));
#7701=CARTESIAN_POINT('',(-3.5,-3.5,4.5));
#7702=CARTESIAN_POINT('Origin',(0.,-3.5,4.5));
#7703=CARTESIAN_POINT('Origin',(0.,-3.5,4.5));
#7704=CARTESIAN_POINT('',(-1.6,-3.5,4.5));
#7705=CARTESIAN_POINT('Origin',(0.,-3.5,4.5));
#7842=UNCERTAINTY_MEASURE_WITH_UNIT(LENGTH_MEASURE(0.001),#7872,
'DISTANCE_ACCURACY_VALUE',
'Maximum model space distance between geometric entities at asserted c
onnectivities');
#7845=UNCERTAINTY_MEASURE_WITH_UNIT(LENGTH_MEASURE(0.001),#7872,
'DISTANCE_ACCURACY_VALUE',
'Maximum model space distance between geometric entities at asserted c
onnectivities');
#7868=(
GEOMETRIC_REPRESENTATION_CONTEXT(3)
GLOBAL_UNCERTAINTY_ASSIGNED_CONTEXT((#7842))
GLOBAL_UNIT_ASSIGNED_CONTEXT((#7872,#7874,#7875))
REPRESENTATION_CONTEXT('','3D')
);
#7871=(
GEOMETRIC_REPRESENTATION_CONTEXT(3)
GLOBAL_UNCERTAINTY_ASSIGNED_CONTEXT((#7845))
GLOBAL_UNIT_ASSIGNED_CONTEXT((#7872,#7874,#7875))
REPRESENTATION_CONTEXT('','3D')
);
#7872=(
LENGTH_UNIT()
NAMED_UNIT(*)
SI_UNIT(.CENTI.,.METRE.)
);
#7874=(
NAMED_UNIT(*)
PLANE_ANGLE_UNIT()
SI_UNIT($,.RADIAN.)
);
#7875=(
NAMED_UNIT(*)
SI_UNIT($,.STERADIAN.)
SOLID_ANGLE_UNIT()
);
#7898=SHAPE_DEFINITION_REPRESENTATION(#7950,#7984);
#7950=PRODUCT_DEFINITION_SHAPE('',$,#8010);
#7984=SHAPE_REPRESENTATION('',(#4809),#7868);
#7987=PRODUCT_DEFINITION_CONTEXT('part definition',#8064,'design');
#8010=PRODUCT_DEFINITION('Drive flange','Drive flange',#8035,#7987);
#8035=PRODUCT_DEFINITION_FORMATION('',$,#8088);
#8064=APPLICATION_CONTEXT(
'Core Data for Automotive Mechanical Design Process');
#8065=PRODUCT_CONTEXT('part definition',#8064,'mechanical');
#8088=PRODUCT('Drive flange','Drive flange','Drive flange',(#8065));
#8140=COLOUR_RGB('Sky Blue',0.24,0.69,0.87);
#8141=FILL_AREA_STYLE_COLOUR('',#8140);
#8142=FILL_AREA_STYLE('',(#8141));
#8143=SURFACE_STYLE_FILL_AREA(#8142);
#8144=SURFACE_SIDE_STYLE('',(#8143));
#8145=SURFACE_STYLE_USAGE(.BOTH.,#8144);
#8146=PRESENTATION_STYLE_ASSIGNMENT((#8145));
ENDSEC;
END-ISO-10303-21;
